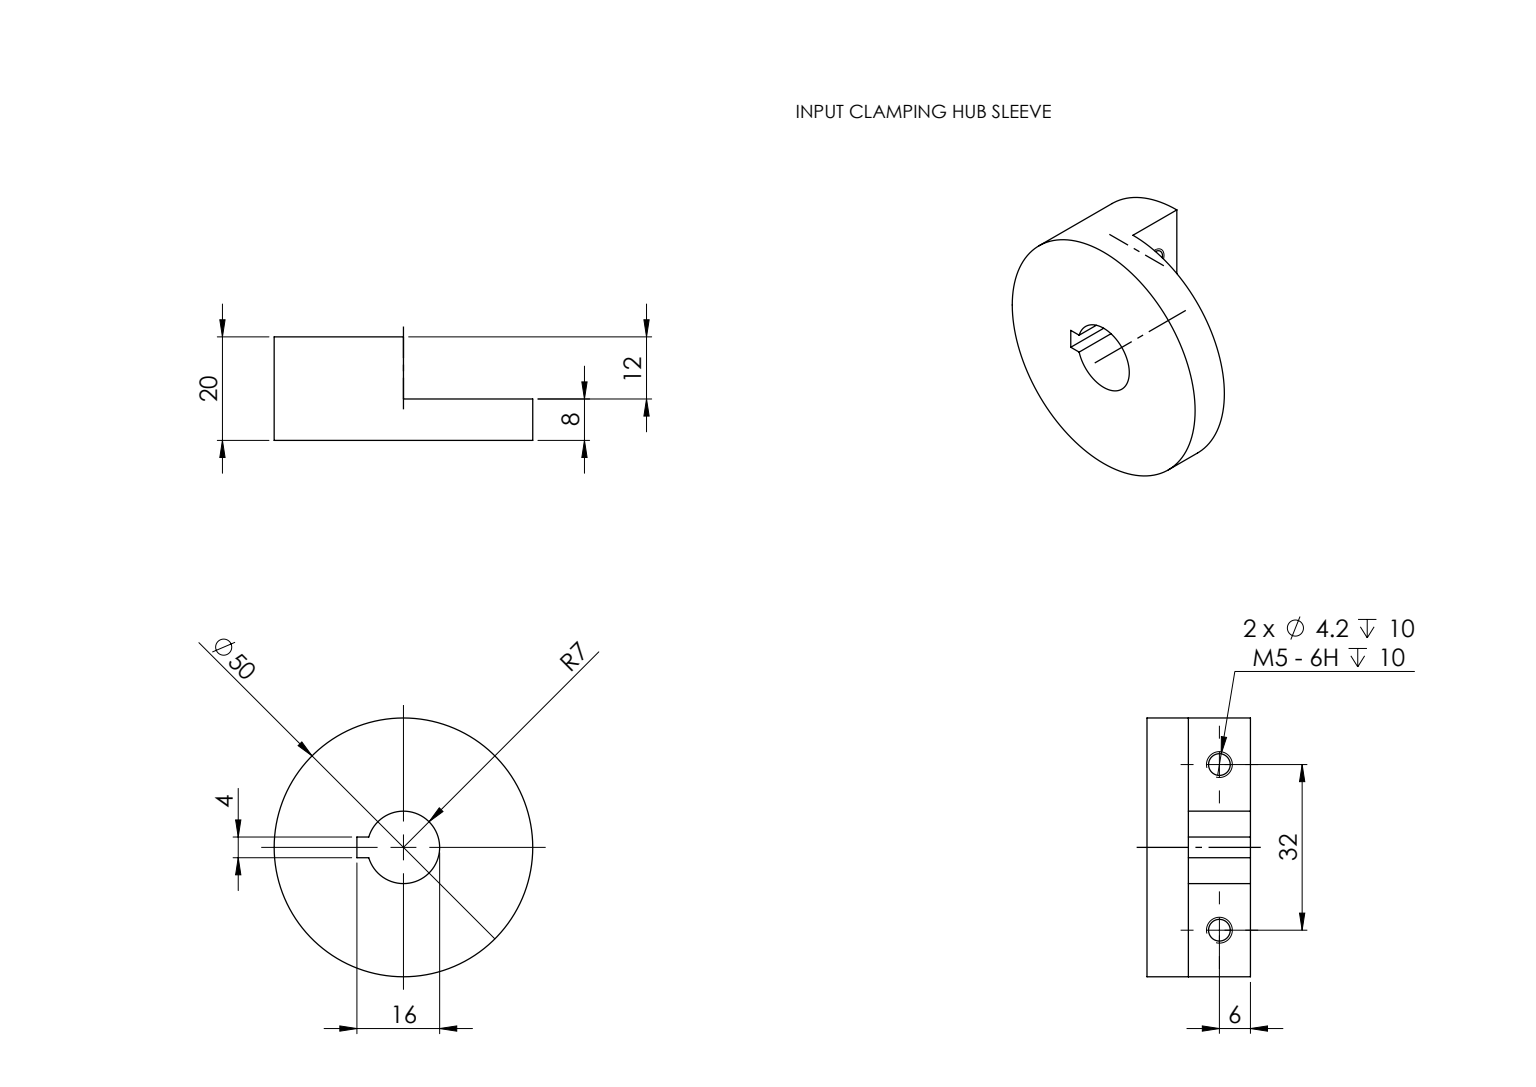
ISO-10303-21;
HEADER;
FILE_DESCRIPTION (('STEP AP214'),
    '1' );
FILE_NAME ('Input Clamping Hub Sleeve.step',
    '2026-10-08T14:09:18',
    ( '' ),
    ( '' ),
    'SwSTEP 2.0',
    'SolidWorks 2026',
    '' );
FILE_SCHEMA (( 'AUTOMOTIVE_DESIGN' ));
ENDSEC;

DATA;
#8=EDGE_CURVE ( 'NONE', #881, #1919, #4427, .T. ) ;
#13=DIRECTION ( 'NONE',  ( -0.000000000000000000, -0.000000000000000000, 1.000000000000000000 ) ) ;
#15=CARTESIAN_POINT ( 'NONE',  ( -6.708203932499367639, 2.000000000000000888, -20.00000000000000000 ) ) ;
#29=DIRECTION ( 'NONE',  ( -0.000000000000000000, -0.000000000000000000, 1.000000000000000000 ) ) ;
#34=FACE_BOUND ( 'NONE', #887, .T. ) ;
#41=LINE ( 'NONE', #2781, #4907 ) ;
#43=DIRECTION ( 'NONE',  ( 1.000000000000000000, -0.000000000000000000, -0.000000000000000000 ) ) ;
#56=DIRECTION ( 'NONE',  ( 0.000000000000000000, 0.000000000000000000, -1.000000000000000000 ) ) ;
#59=ORIENTED_EDGE ( 'NONE', *, *, #2870, .T. ) ;
#63=DIRECTION ( 'NONE',  ( 1.000000000000000000, -0.000000000000000000, 0.000000000000000000 ) ) ;
#66=ORIENTED_EDGE ( 'NONE', *, *, #2378, .T. ) ;
#73=DIRECTION ( 'NONE',  ( 1.000000000000000000, -0.000000000000000000, -0.000000000000000000 ) ) ;
#80=DIRECTION ( 'NONE',  ( -0.000000000000000000, -0.000000000000000000, 1.000000000000000000 ) ) ;
#87=DIRECTION ( 'NONE',  ( 1.357798298438996130E-15, -1.000000000000000000, 0.000000000000000000 ) ) ;
#91=CIRCLE ( 'NONE', #3370, 2.099999999999997868 ) ;
#94=DIRECTION ( 'NONE',  ( -1.000000000000000000, 0.000000000000000000, 0.000000000000000000 ) ) ;
#105=FACE_OUTER_BOUND ( 'NONE', #4278, .T. ) ;
#107=VERTEX_POINT ( 'NONE', #3557 ) ;
#111=CARTESIAN_POINT ( 'NONE',  ( -9.000000000000003553, -1.999999999999999112, -20.00000000000000000 ) ) ;
#117=CARTESIAN_POINT ( 'NONE',  ( 0.000000000000000000, 25.00000000000000000, -20.00000000000000000 ) ) ;
#132=DIRECTION ( 'NONE',  ( 1.000000000000000000, 2.168404344971009361E-16, 0.000000000000000000 ) ) ;
#136=EDGE_LOOP ( 'NONE', ( #1667, #4376 ) ) ;
#140=DIRECTION ( 'NONE',  ( 0.000000000000000000, 0.000000000000000000, -1.000000000000000000 ) ) ;
#147=CARTESIAN_POINT ( 'NONE',  ( 0.000000000000000000, 0.000000000000000000, -20.00000000000000000 ) ) ;
#149=CARTESIAN_POINT ( 'NONE',  ( -9.999999999999975131, -16.00000000000000000, -28.10000000000000142 ) ) ;
#153=VERTEX_POINT ( 'NONE', #3959 ) ;
#157=ORIENTED_EDGE ( 'NONE', *, *, #1693, .F. ) ;
#166=EDGE_CURVE ( 'NONE', #107, #941, #3578, .T. ) ;
#173=VECTOR ( 'NONE', #4086, 1000.000000000000000 ) ;
#208=ADVANCED_FACE ( 'NONE', ( #2082 ), #4946, .F. ) ;
#223=CARTESIAN_POINT ( 'NONE',  ( -7.332110811570578784E-14, -6.999999999999999112, -32.00000000000000000 ) ) ;
#231=CARTESIAN_POINT ( 'NONE',  ( 2.444036937190193033E-14, 6.999999999999999112, -20.00000000000000000 ) ) ;
#240=VERTEX_POINT ( 'NONE', #2913 ) ;
#241=ORIENTED_EDGE ( 'NONE', *, *, #4762, .F. ) ;
#243=LINE ( 'NONE', #1762, #4071 ) ;
#248=LINE ( 'NONE', #4070, #1913 ) ;
#259=DIRECTION ( 'NONE',  ( 0.000000000000000000, 0.000000000000000000, -1.000000000000000000 ) ) ;
#270=FACE_OUTER_BOUND ( 'NONE', #2121, .T. ) ;
#275=MECHANICAL_DESIGN_GEOMETRIC_PRESENTATION_REPRESENTATION('',(#1381),#2264);
#281=DIRECTION ( 'NONE',  ( 0.000000000000000000, 0.000000000000000000, -1.000000000000000000 ) ) ;
#289=CARTESIAN_POINT ( 'NONE',  ( -9.000000000000003553, -1.999999999999999112, -32.00000000000000000 ) ) ;
#300=DIRECTION ( 'NONE',  ( 0.000000000000000000, 0.000000000000000000, -1.000000000000000000 ) ) ;
#303=ORIENTED_EDGE ( 'NONE', *, *, #3258, .T. ) ;
#305=( GEOMETRIC_REPRESENTATION_CONTEXT ( 3 ) GLOBAL_UNCERTAINTY_ASSIGNED_CONTEXT ( ( #1895 ) ) GLOBAL_UNIT_ASSIGNED_CONTEXT ( ( #3470, #4642, #2320 ) ) REPRESENTATION_CONTEXT ( 'NONE', 'WORKASPACE' ) );
#314=CARTESIAN_POINT ( 'NONE',  ( 0.000000000000000000, 0.000000000000000000, -32.00000000000000000 ) ) ;
#322=EDGE_CURVE ( 'NONE', #2990, #2143, #2362, .T. ) ;
#327=CIRCLE ( 'NONE', #3446, 2.099999999999990763 ) ;
#335=CYLINDRICAL_SURFACE ( 'NONE', #4166, 25.00000000000000000 ) ;
#338=DIRECTION ( 'NONE',  ( 0.000000000000000000, 0.000000000000000000, -1.000000000000000000 ) ) ;
#345=ADVANCED_BREP_SHAPE_REPRESENTATION ( '', ( #3609, #1918 ), #305 ) ;
#349=ORIENTED_EDGE ( 'NONE', *, *, #1643, .T. ) ;
#361=AXIS2_PLACEMENT_3D ( 'NONE', #2287, #1500, #3043 ) ;
#362=EDGE_CURVE ( 'NONE', #1707, #1968, #2444, .T. ) ;
#369=CARTESIAN_POINT ( 'NONE',  ( -9.999999999999975131, -16.00000000000000000, -28.10000000000000142 ) ) ;
#370=CARTESIAN_POINT ( 'NONE',  ( 0.000000000000000000, 0.000000000000000000, -32.00000000000000000 ) ) ;
#377=CARTESIAN_POINT ( 'NONE',  ( -6.708203932499367639, 2.000000000000000888, -12.00000000000000000 ) ) ;
#380=ORIENTED_EDGE ( 'NONE', *, *, #2599, .F. ) ;
#386=ADVANCED_FACE ( 'NONE', ( #971 ), #1098, .T. ) ;
#398=VERTEX_POINT ( 'NONE', #2707 ) ;
#410=DIRECTION ( 'NONE',  ( 0.000000000000000000, 0.000000000000000000, -1.000000000000000000 ) ) ;
#414=CONICAL_SURFACE ( 'NONE', #1848, 2.099999999999997868, 1.029744258676653423 ) ;
#423=CARTESIAN_POINT ( 'NONE',  ( 6.999999999999999112, 0.000000000000000000, -20.00000000000000000 ) ) ;
#432=AXIS2_PLACEMENT_3D ( 'NONE', #1311, #2846, #832 ) ;
#452=PRESENTATION_STYLE_ASSIGNMENT (( #3871 ) ) ;
#459=DIRECTION ( 'NONE',  ( 1.000000000000000000, -0.000000000000000000, -0.000000000000000000 ) ) ;
#465=FILL_AREA_STYLE_COLOUR ( '', #4492 ) ;
#467=VERTEX_POINT ( 'NONE', #1823 ) ;
#468=VERTEX_POINT ( 'NONE', #3797 ) ;
#487=EDGE_CURVE ( 'NONE', #468, #1707, #3426, .T. ) ;
#504=EDGE_LOOP ( 'NONE', ( #3356, #2233, #3231, #687, #2325, #2539 ) ) ;
#506=VECTOR ( 'NONE', #1907, 1000.000000000000000 ) ;
#527=CARTESIAN_POINT ( 'NONE',  ( 0.000000000000000000, -1.999999999999999112, -12.00000000000000000 ) ) ;
#531=CARTESIAN_POINT ( 'NONE',  ( -7.332110811570578784E-14, -6.999999999999999112, -20.00000000000000000 ) ) ;
#532=CARTESIAN_POINT ( 'NONE',  ( -9.999999999999975131, -16.00000000000000000, -26.00000000000000355 ) ) ;
#538=DIRECTION ( 'NONE',  ( 0.000000000000000000, 0.000000000000000000, -1.000000000000000000 ) ) ;
#541=EDGE_CURVE ( 'NONE', #4479, #4279, #1671, .T. ) ;
#557=ORIENTED_EDGE ( 'NONE', *, *, #3777, .T. ) ;
#559=CARTESIAN_POINT ( 'NONE',  ( 0.000000000000000000, 25.00000000000000000, -32.00000000000000000 ) ) ;
#574=PRODUCT_CONTEXT ( 'NONE', #3334, 'mechanical' ) ;
#577=ORIENTED_EDGE ( 'NONE', *, *, #1279, .T. ) ;
#582=CYLINDRICAL_SURFACE ( 'NONE', #2017, 25.00000000000000000 ) ;
#583=AXIS2_PLACEMENT_3D ( 'NONE', #4630, #73, #1654 ) ;
#594=AXIS2_PLACEMENT_3D ( 'NONE', #1405, #1084, #1809 ) ;
#601=EDGE_CURVE ( 'NONE', #4279, #3704, #1126, .T. ) ;
#610=DIRECTION ( 'NONE',  ( 0.5150380749100550437, 0.000000000000000000, -0.8571673007021117785 ) ) ;
#622=ADVANCED_FACE ( 'NONE', ( #3955 ), #3927, .F. ) ;
#623=EDGE_CURVE ( 'NONE', #4219, #2953, #1516, .T. ) ;
#625=FACE_BOUND ( 'NONE', #874, .T. ) ;
#646=EDGE_CURVE ( 'NONE', #1680, #4219, #2359, .T. ) ;
#670=AXIS2_PLACEMENT_3D ( 'NONE', #3868, #3890, #1940 ) ;
#687=ORIENTED_EDGE ( 'NONE', *, *, #2074, .F. ) ;
#711=CARTESIAN_POINT ( 'NONE',  ( 0.000000000000000000, 0.000000000000000000, -20.00000000000000000 ) ) ;
#714=ORIENTED_EDGE ( 'NONE', *, *, #623, .F. ) ;
#723=CARTESIAN_POINT ( 'NONE',  ( -9.000000000000003553, -1.999999999999999112, -32.00000000000000000 ) ) ;
#729=ORIENTED_EDGE ( 'NONE', *, *, #2155, .T. ) ;
#733=LINE ( 'NONE', #3464, #4106 ) ;
#737=AXIS2_PLACEMENT_3D ( 'NONE', #2501, #946, #4021 ) ;
#738=VECTOR ( 'NONE', #1161, 1000.000000000000000 ) ;
#741=CARTESIAN_POINT ( 'NONE',  ( -9.000000000000003553, -1.999999999999999112, -12.00000000000000000 ) ) ;
#744=ORIENTED_EDGE ( 'NONE', *, *, #487, .T. ) ;
#752=DIRECTION ( 'NONE',  ( -1.000000000000000000, 0.000000000000000000, 0.000000000000000000 ) ) ;
#761=EDGE_LOOP ( 'NONE', ( #2798, #4883, #1651, #3117 ) ) ;
#762=DIRECTION ( 'NONE',  ( 1.000000000000000000, -0.000000000000000000, -0.000000000000000000 ) ) ;
#771=CARTESIAN_POINT ( 'NONE',  ( -25.00000000000000000, 3.061616997868383043E-15, -12.00000000000000000 ) ) ;
#779=CARTESIAN_POINT ( 'NONE',  ( -10.00000000000002132, 16.00000000000000000, -26.00000000000000355 ) ) ;
#780=CARTESIAN_POINT ( 'NONE',  ( -10.00000000000002132, 16.00000000000000000, -26.00000000000000355 ) ) ;
#788=CYLINDRICAL_SURFACE ( 'NONE', #4749, 2.099999999999994316 ) ;
#791=CARTESIAN_POINT ( 'NONE',  ( 2.172477277502393807E-14, -16.00000000000000000, -28.09999999999999787 ) ) ;
#792=DIRECTION ( 'NONE',  ( -0.000000000000000000, -0.000000000000000000, 1.000000000000000000 ) ) ;
#814=FILL_AREA_STYLE ('',( #4620 ) ) ;
#818=LINE ( 'NONE', #117, #4015 ) ;
#825=DIRECTION ( 'NONE',  ( 0.000000000000000000, 0.000000000000000000, -1.000000000000000000 ) ) ;
#832=DIRECTION ( 'NONE',  ( 1.000000000000000000, 0.000000000000000000, 0.000000000000000000 ) ) ;
#834=ORIENTED_EDGE ( 'NONE', *, *, #848, .T. ) ;
#841=VECTOR ( 'NONE', #3213, 1000.000000000000000 ) ;
#842=ORIENTED_EDGE ( 'NONE', *, *, #1820, .T. ) ;
#843=ORIENTED_EDGE ( 'NONE', *, *, #4547, .T. ) ;
#844=DIRECTION ( 'NONE',  ( 1.000000000000000000, -0.000000000000000000, -0.000000000000000000 ) ) ;
#848=EDGE_CURVE ( 'NONE', #3754, #468, #3922, .T. ) ;
#853=PRODUCT ( 'Input Clamping Hub Sleeve', 'Input Clamping Hub Sleeve', '', ( #574 ) ) ;
#856=SURFACE_SIDE_STYLE ('',( #2768 ) ) ;
#874=EDGE_LOOP ( 'NONE', ( #4323, #3014, #1256, #4847, #349 ) ) ;
#875=ORIENTED_EDGE ( 'NONE', *, *, #1061, .F. ) ;
#881=VERTEX_POINT ( 'NONE', #3443 ) ;
#883=ORIENTED_EDGE ( 'NONE', *, *, #3777, .F. ) ;
#887=EDGE_LOOP ( 'NONE', ( #157, #875 ) ) ;
#888=AXIS2_PLACEMENT_3D ( 'NONE', #1755, #1321, #140 ) ;
#894=VERTEX_POINT ( 'NONE', #741 ) ;
#898=EDGE_CURVE ( 'NONE', #3704, #1580, #4887, .T. ) ;
#900=AXIS2_PLACEMENT_3D ( 'NONE', #1114, #4163, #1487 ) ;
#912=ORIENTED_EDGE ( 'NONE', *, *, #4390, .F. ) ;
#919=ORIENTED_EDGE ( 'NONE', *, *, #1536, .F. ) ;
#926=ORIENTED_EDGE ( 'NONE', *, *, #2599, .T. ) ;
#930=EDGE_CURVE ( 'NONE', #153, #1150, #1071, .T. ) ;
#941=VERTEX_POINT ( 'NONE', #369 ) ;
#946=DIRECTION ( 'NONE',  ( 1.000000000000000000, -0.000000000000000000, -0.000000000000000000 ) ) ;
#953=ORIENTED_EDGE ( 'NONE', *, *, #646, .F. ) ;
#957=AXIS2_PLACEMENT_3D ( 'NONE', #1468, #300, #2156 ) ;
#971=FACE_OUTER_BOUND ( 'NONE', #761, .T. ) ;
#975=AXIS2_PLACEMENT_3D ( 'NONE', #1315, #3964, #538 ) ;
#976=( LENGTH_UNIT ( ) NAMED_UNIT ( * ) SI_UNIT ( .MILLI., .METRE. ) );
#1001=DIRECTION ( 'NONE',  ( 0.000000000000000000, 0.000000000000000000, -1.000000000000000000 ) ) ;
#1004=( NAMED_UNIT ( * ) SI_UNIT ( $, .STERADIAN. ) SOLID_ANGLE_UNIT ( ) );
#1008=EDGE_LOOP ( 'NONE', ( #4046, #1246, #577 ) ) ;
#1020=EDGE_LOOP ( 'NONE', ( #1983, #557, #59, #4058, #714, #953 ) ) ;
#1045=AXIS2_PLACEMENT_3D ( 'NONE', #711, #2978, #4541 ) ;
#1046=LINE ( 'NONE', #2578, #4876 ) ;
#1052=AXIS2_PLACEMENT_3D ( 'NONE', #4364, #259, #3986 ) ;
#1061=EDGE_CURVE ( 'NONE', #1150, #2856, #327, .T. ) ;
#1068=CIRCLE ( 'NONE', #3623, 6.999999999999999112 ) ;
#1071=LINE ( 'NONE', #2271, #2733 ) ;
#1084=DIRECTION ( 'NONE',  ( 0.000000000000000000, 0.000000000000000000, -1.000000000000000000 ) ) ;
#1092=CYLINDRICAL_SURFACE ( 'NONE', #900, 6.999999999999999112 ) ;
#1093=DIRECTION ( 'NONE',  ( -0.000000000000000000, -0.000000000000000000, 1.000000000000000000 ) ) ;
#1098=PLANE ( 'NONE',  #1638 ) ;
#1114=CARTESIAN_POINT ( 'NONE',  ( 0.000000000000000000, 0.000000000000000000, -20.00000000000000000 ) ) ;
#1115=DIRECTION ( 'NONE',  ( 1.000000000000000000, 0.000000000000000000, 0.000000000000000000 ) ) ;
#1119=ORIENTED_EDGE ( 'NONE', *, *, #4580, .F. ) ;
#1125=ORIENTED_EDGE ( 'NONE', *, *, #3211, .T. ) ;
#1126=CIRCLE ( 'NONE', #4884, 6.999999999999999112 ) ;
#1127=CONICAL_SURFACE ( 'NONE', #3765, 2.099999999999997868, 1.029744258676653423 ) ;
#1133=EDGE_LOOP ( 'NONE', ( #1119, #2771, #3567, #1730 ) ) ;
#1146=CARTESIAN_POINT ( 'NONE',  ( 0.000000000000000000, 0.000000000000000000, 0.000000000000000000 ) ) ;
#1150=VERTEX_POINT ( 'NONE', #3180 ) ;
#1159=DIRECTION ( 'NONE',  ( 0.000000000000000000, 0.000000000000000000, -1.000000000000000000 ) ) ;
#1160=CARTESIAN_POINT ( 'NONE',  ( 2.302289838212012812E-14, -16.00000000000000000, -26.00000000000000355 ) ) ;
#1161=DIRECTION ( 'NONE',  ( -0.000000000000000000, -0.000000000000000000, 1.000000000000000000 ) ) ;
#1181=PRODUCT_DEFINITION ( 'UNKNOWN', '', #4711, #3035 ) ;
#1183=CYLINDRICAL_SURFACE ( 'NONE', #4656, 2.099999999999994316 ) ;
#1185=LINE ( 'NONE', #1931, #738 ) ;
#1193=ORIENTED_EDGE ( 'NONE', *, *, #2053, .T. ) ;
#1198=ORIENTED_EDGE ( 'NONE', *, *, #2102, .T. ) ;
#1200=DIRECTION ( 'NONE',  ( -1.000000000000000000, 0.000000000000000000, 0.000000000000000000 ) ) ;
#1222=VECTOR ( 'NONE', #4199, 1000.000000000000000 ) ;
#1231=ORIENTED_EDGE ( 'NONE', *, *, #1820, .F. ) ;
#1235=FILL_AREA_STYLE ('',( #465 ) ) ;
#1243=CARTESIAN_POINT ( 'NONE',  ( 0.000000000000000000, -25.00000000000000000, -20.00000000000000000 ) ) ;
#1246=ORIENTED_EDGE ( 'NONE', *, *, #166, .T. ) ;
#1252=ORIENTED_EDGE ( 'NONE', *, *, #8, .T. ) ;
#1256=ORIENTED_EDGE ( 'NONE', *, *, #2102, .F. ) ;
#1279=EDGE_CURVE ( 'NONE', #941, #467, #3055, .T. ) ;
#1288=FACE_OUTER_BOUND ( 'NONE', #2721, .T. ) ;
#1290=ORIENTED_EDGE ( 'NONE', *, *, #4955, .T. ) ;
#1311=CARTESIAN_POINT ( 'NONE',  ( 0.000000000000000000, 0.000000000000000000, -20.00000000000000000 ) ) ;
#1315=CARTESIAN_POINT ( 'NONE',  ( -2.042664716792774803E-14, 16.00000000000000000, -26.00000000000000355 ) ) ;
#1317=CARTESIAN_POINT ( 'NONE',  ( -9.000000000000001776, 3.903127820947817540E-15, -20.00000000000000000 ) ) ;
#1321=DIRECTION ( 'NONE',  ( 1.000000000000000000, -0.000000000000000000, -0.000000000000000000 ) ) ;
#1331=SHAPE_DEFINITION_REPRESENTATION ( #1603, #2032 ) ;
#1347=DIRECTION ( 'NONE',  ( -1.000000000000000000, 0.000000000000000000, 0.000000000000000000 ) ) ;
#1350=FACE_OUTER_BOUND ( 'NONE', #1431, .T. ) ;
#1351=VECTOR ( 'NONE', #2106, 1000.000000000000000 ) ;
#1358=CARTESIAN_POINT ( 'NONE',  ( -10.00000000000002132, 16.00000000000000000, -28.10000000000000142 ) ) ;
#1361=EDGE_CURVE ( 'NONE', #3396, #3754, #4924, .T. ) ;
#1379=CARTESIAN_POINT ( 'NONE',  ( 0.000000000000000000, 0.000000000000000000, -32.00000000000000000 ) ) ;
#1381=STYLED_ITEM ( 'NONE', ( #2956 ), #3609 ) ;
#1383=ORIENTED_EDGE ( 'NONE', *, *, #2555, .F. ) ;
#1388=LINE ( 'NONE', #1358, #4480 ) ;
#1401=CARTESIAN_POINT ( 'NONE',  ( -9.999999999999975131, -16.00000000000000000, -26.00000000000000355 ) ) ;
#1405=CARTESIAN_POINT ( 'NONE',  ( 0.000000000000000000, 0.000000000000000000, -12.00000000000000000 ) ) ;
#1406=DIRECTION ( 'NONE',  ( -0.000000000000000000, -0.000000000000000000, 1.000000000000000000 ) ) ;
#1418=CARTESIAN_POINT ( 'NONE',  ( -2.172477277502393807E-14, 16.00000000000000000, -26.00000000000000355 ) ) ;
#1420=ADVANCED_FACE ( 'NONE', ( #2595 ), #335, .T. ) ;
#1431=EDGE_LOOP ( 'NONE', ( #303, #1383, #4360, #843 ) ) ;
#1432=FACE_OUTER_BOUND ( 'NONE', #4960, .T. ) ;
#1435=VECTOR ( 'NONE', #792, 1000.000000000000000 ) ;
#1456=ORIENTED_EDGE ( 'NONE', *, *, #4572, .T. ) ;
#1463=DIRECTION ( 'NONE',  ( -4.336808689942018722E-16, -1.000000000000000000, 0.000000000000000000 ) ) ;
#1468=CARTESIAN_POINT ( 'NONE',  ( 0.000000000000000000, 0.000000000000000000, -20.00000000000000000 ) ) ;
#1483=DIRECTION ( 'NONE',  ( 0.000000000000000000, 0.000000000000000000, -1.000000000000000000 ) ) ;
#1485=ADVANCED_FACE ( 'NONE', ( #3413 ), #414, .F. ) ;
#1487=DIRECTION ( 'NONE',  ( 1.000000000000000000, 0.000000000000000000, 0.000000000000000000 ) ) ;
#1489=ORIENTED_EDGE ( 'NONE', *, *, #166, .F. ) ;
#1497=CARTESIAN_POINT ( 'NONE',  ( -2.042664716792774803E-14, 16.00000000000000000, -28.09999999999999432 ) ) ;
#1500=DIRECTION ( 'NONE',  ( 0.000000000000000000, -1.000000000000000000, 0.000000000000000000 ) ) ;
#1502=DIRECTION ( 'NONE',  ( 0.000000000000000000, 0.000000000000000000, -1.000000000000000000 ) ) ;
#1506=CARTESIAN_POINT ( 'NONE',  ( -9.000000000000001776, 3.903127820947817540E-15, -12.00000000000000000 ) ) ;
#1510=EDGE_CURVE ( 'NONE', #3209, #153, #1610, .T. ) ;
#1516=CIRCLE ( 'NONE', #3756, 25.00000000000000000 ) ;
#1524=LINE ( 'NONE', #3785, #3614 ) ;
#1536=EDGE_CURVE ( 'NONE', #240, #153, #3462, .T. ) ;
#1541=DIRECTION ( 'NONE',  ( -0.000000000000000000, -0.000000000000000000, 1.000000000000000000 ) ) ;
#1560=DIRECTION ( 'NONE',  ( 1.000000000000000000, -0.000000000000000000, -0.000000000000000000 ) ) ;
#1561=DIRECTION ( 'NONE',  ( 0.000000000000000000, 0.000000000000000000, -1.000000000000000000 ) ) ;
#1572=ORIENTED_EDGE ( 'NONE', *, *, #4762, .T. ) ;
#1580=VERTEX_POINT ( 'NONE', #2392 ) ;
#1582=DIRECTION ( 'NONE',  ( 1.000000000000000000, -0.000000000000000000, -0.000000000000000000 ) ) ;
#1584=PLANE ( 'NONE',  #670 ) ;
#1593=AXIS2_PLACEMENT_3D ( 'NONE', #1418, #2954, #3772 ) ;
#1603=PRODUCT_DEFINITION_SHAPE ( 'NONE', 'NONE',  #1181 ) ;
#1610=CIRCLE ( 'NONE', #1928, 2.099999999999997868 ) ;
#1618=PLANE ( 'NONE',  #2668 ) ;
#1619=CARTESIAN_POINT ( 'NONE',  ( -6.708203932499366751, -2.000000000000003553, -32.00000000000000000 ) ) ;
#1626=ORIENTED_EDGE ( 'NONE', *, *, #2155, .F. ) ;
#1634=CARTESIAN_POINT ( 'NONE',  ( -10.00000000000002132, 16.00000000000000000, -23.90000000000000568 ) ) ;
#1635=CARTESIAN_POINT ( 'NONE',  ( -9.999999999999975131, -16.00000000000000000, -23.90000000000000568 ) ) ;
#1638=AXIS2_PLACEMENT_3D ( 'NONE', #4574, #4124, #3744 ) ;
#1642=FACE_OUTER_BOUND ( 'NONE', #2000, .T. ) ;
#1643=EDGE_CURVE ( 'NONE', #4802, #2990, #2695, .T. ) ;
#1651=ORIENTED_EDGE ( 'NONE', *, *, #4474, .F. ) ;
#1654=DIRECTION ( 'NONE',  ( 0.000000000000000000, 0.000000000000000000, -1.000000000000000000 ) ) ;
#1661=MECHANICAL_DESIGN_GEOMETRIC_PRESENTATION_REPRESENTATION('',(#4381),#4055);
#1665=FACE_BOUND ( 'NONE', #136, .T. ) ;
#1667=ORIENTED_EDGE ( 'NONE', *, *, #2961, .F. ) ;
#1671=LINE ( 'NONE', #3523, #2089 ) ;
#1680=VERTEX_POINT ( 'NONE', #559 ) ;
#1682=AXIS2_PLACEMENT_3D ( 'NONE', #532, #459, #2057 ) ;
#1693=EDGE_CURVE ( 'NONE', #2856, #1150, #2104, .T. ) ;
#1699=CIRCLE ( 'NONE', #737, 2.099999999999990763 ) ;
#1701=VECTOR ( 'NONE', #1541, 1000.000000000000000 ) ;
#1707=VERTEX_POINT ( 'NONE', #4770 ) ;
#1710=PLANE ( 'NONE',  #4164 ) ;
#1719=ORIENTED_EDGE ( 'NONE', *, *, #1693, .T. ) ;
#1725=ADVANCED_FACE ( 'NONE', ( #2917 ), #3632, .T. ) ;
#1730=ORIENTED_EDGE ( 'NONE', *, *, #2961, .T. ) ;
#1737=CYLINDRICAL_SURFACE ( 'NONE', #2828, 2.099999999999994316 ) ;
#1749=VECTOR ( 'NONE', #4469, 1000.000000000000000 ) ;
#1752=AXIS2_PLACEMENT_3D ( 'NONE', #3724, #13, #4466 ) ;
#1755=CARTESIAN_POINT ( 'NONE',  ( -9.999999999999975131, -16.00000000000000000, -26.00000000000000355 ) ) ;
#1762=CARTESIAN_POINT ( 'NONE',  ( 25.00000000000000000, 0.000000000000000000, -20.00000000000000000 ) ) ;
#1763=VECTOR ( 'NONE', #80, 1000.000000000000000 ) ;
#1766=EDGE_LOOP ( 'NONE', ( #380, #3790, #3447, #3166 ) ) ;
#1785=CARTESIAN_POINT ( 'NONE',  ( -9.999999999999975131, -16.00000000000000000, -26.00000000000000355 ) ) ;
#1809=DIRECTION ( 'NONE',  ( -1.000000000000000000, 0.000000000000000000, 0.000000000000000000 ) ) ;
#1820=EDGE_CURVE ( 'NONE', #467, #941, #3375, .T. ) ;
#1823=CARTESIAN_POINT ( 'NONE',  ( -9.999999999999975131, -16.00000000000000000, -23.90000000000000568 ) ) ;
#1826=DIRECTION ( 'NONE',  ( 1.000000000000000000, -0.000000000000000000, -0.000000000000000000 ) ) ;
#1833=ORIENTED_EDGE ( 'NONE', *, *, #1510, .F. ) ;
#1848=AXIS2_PLACEMENT_3D ( 'NONE', #1785, #1560, #410 ) ;
#1854=DIRECTION ( 'NONE',  ( 1.000000000000000000, -0.000000000000000000, -0.000000000000000000 ) ) ;
#1861=DIRECTION ( 'NONE',  ( 1.000000000000000000, 0.000000000000000000, 0.000000000000000000 ) ) ;
#1895=UNCERTAINTY_MEASURE_WITH_UNIT (LENGTH_MEASURE( 1.000000000000000082E-05 ), #3470, 'distance_accuracy_value', 'NONE');
#1907=DIRECTION ( 'NONE',  ( 0.5150380749100550437, 1.049727191138617956E-16, 0.8571673007021117785 ) ) ;
#1913=VECTOR ( 'NONE', #3743, 1000.000000000000000 ) ;
#1918=AXIS2_PLACEMENT_3D ( 'NONE', #1146, #2700, #1115 ) ;
#1919=VERTEX_POINT ( 'NONE', #771 ) ;
#1928=AXIS2_PLACEMENT_3D ( 'NONE', #779, #1582, #56 ) ;
#1931=CARTESIAN_POINT ( 'NONE',  ( 6.999999999999999112, 0.000000000000000000, -20.00000000000000000 ) ) ;
#1932=ORIENTED_EDGE ( 'NONE', *, *, #4474, .T. ) ;
#1933=CIRCLE ( 'NONE', #4653, 25.00000000000000000 ) ;
#1935=EDGE_CURVE ( 'NONE', #3401, #3396, #4280, .T. ) ;
#1940=DIRECTION ( 'NONE',  ( 1.357798298438996130E-15, -1.000000000000000000, 0.000000000000000000 ) ) ;
#1948=DIRECTION ( 'NONE',  ( 1.000000000000000000, -0.000000000000000000, -0.000000000000000000 ) ) ;
#1968=VERTEX_POINT ( 'NONE', #2083 ) ;
#1977=ORIENTED_EDGE ( 'NONE', *, *, #4367, .F. ) ;
#1983=ORIENTED_EDGE ( 'NONE', *, *, #3211, .F. ) ;
#2000=EDGE_LOOP ( 'NONE', ( #1572, #3081, #2766, #1193 ) ) ;
#2017=AXIS2_PLACEMENT_3D ( 'NONE', #2890, #4404, #3193 ) ;
#2024=AXIS2_PLACEMENT_3D ( 'NONE', #1401, #1826, #2936 ) ;
#2029=AXIS2_PLACEMENT_3D ( 'NONE', #370, #3373, #4543 ) ;
#2032=SHAPE_REPRESENTATION ( 'Input Clamping Hub Sleeve', ( #1918 ), #305 ) ;
#2053=EDGE_CURVE ( 'NONE', #468, #1580, #3671, .T. ) ;
#2055=CARTESIAN_POINT ( 'NONE',  ( -10.00000000000002132, 16.00000000000000000, -28.10000000000000142 ) ) ;
#2057=DIRECTION ( 'NONE',  ( 0.000000000000000000, 0.000000000000000000, -1.000000000000000000 ) ) ;
#2062=FACE_OUTER_BOUND ( 'NONE', #504, .T. ) ;
#2066=EDGE_CURVE ( 'NONE', #4479, #398, #4900, .T. ) ;
#2074=EDGE_CURVE ( 'NONE', #398, #2990, #3445, .T. ) ;
#2082=FACE_OUTER_BOUND ( 'NONE', #2337, .T. ) ;
#2083=CARTESIAN_POINT ( 'NONE',  ( -25.00000000000000000, 3.061616997868383043E-15, -32.00000000000000000 ) ) ;
#2089=VECTOR ( 'NONE', #2785, 1000.000000000000000 ) ;
#2102=EDGE_CURVE ( 'NONE', #894, #2727, #2758, .T. ) ;
#2104=CIRCLE ( 'NONE', #975, 2.099999999999990763 ) ;
#2106=DIRECTION ( 'NONE',  ( 4.073394895316987600E-15, -1.000000000000000000, 0.000000000000000000 ) ) ;
#2121=EDGE_LOOP ( 'NONE', ( #241, #4188, #2234, #1626, #4386, #1456 ) ) ;
#2128=FACE_OUTER_BOUND ( 'NONE', #4827, .T. ) ;
#2143=VERTEX_POINT ( 'NONE', #2832 ) ;
#2155=EDGE_CURVE ( 'NONE', #4219, #4279, #818, .T. ) ;
#2156=DIRECTION ( 'NONE',  ( -1.000000000000000000, 0.000000000000000000, 0.000000000000000000 ) ) ;
#2160=ADVANCED_FACE ( 'NONE', ( #1665, #1642 ), #1618, .F. ) ;
#2194=DIRECTION ( 'NONE',  ( 1.000000000000000000, -0.000000000000000000, -0.000000000000000000 ) ) ;
#2209=DIRECTION ( 'NONE',  ( -0.000000000000000000, -0.000000000000000000, 1.000000000000000000 ) ) ;
#2219=PLANE ( 'NONE',  #2995 ) ;
#2231=CARTESIAN_POINT ( 'NONE',  ( -9.000000000000001776, 2.000000000000000000, -32.00000000000000000 ) ) ;
#2233=ORIENTED_EDGE ( 'NONE', *, *, #4390, .T. ) ;
#2234=ORIENTED_EDGE ( 'NONE', *, *, #601, .F. ) ;
#2253=EDGE_CURVE ( 'NONE', #240, #3209, #1388, .T. ) ;
#2264=( GEOMETRIC_REPRESENTATION_CONTEXT ( 3 ) GLOBAL_UNCERTAINTY_ASSIGNED_CONTEXT ( ( #4545 ) ) GLOBAL_UNIT_ASSIGNED_CONTEXT ( ( #976, #3281, #1004 ) ) REPRESENTATION_CONTEXT ( 'NONE', 'WORKASPACE' ) );
#2266=CARTESIAN_POINT ( 'NONE',  ( -10.00000000000002132, 16.00000000000000000, -26.00000000000000355 ) ) ;
#2271=CARTESIAN_POINT ( 'NONE',  ( -2.172477277502393807E-14, 16.00000000000000000, -23.90000000000000924 ) ) ;
#2287=CARTESIAN_POINT ( 'NONE',  ( 0.000000000000000000, -1.999999999999999112, -20.00000000000000000 ) ) ;
#2313=LINE ( 'NONE', #111, #1763 ) ;
#2320=( NAMED_UNIT ( * ) SI_UNIT ( $, .STERADIAN. ) SOLID_ANGLE_UNIT ( ) );
#2325=ORIENTED_EDGE ( 'NONE', *, *, #2066, .F. ) ;
#2337=EDGE_LOOP ( 'NONE', ( #1198, #1977, #3574, #2996 ) ) ;
#2348=SURFACE_SIDE_STYLE ('',( #4930 ) ) ;
#2359=LINE ( 'NONE', #4277, #1435 ) ;
#2362=CIRCLE ( 'NONE', #4759, 6.999999999999999112 ) ;
#2371=FACE_OUTER_BOUND ( 'NONE', #3969, .T. ) ;
#2378=EDGE_CURVE ( 'NONE', #1707, #2498, #3735, .T. ) ;
#2392=CARTESIAN_POINT ( 'NONE',  ( -3.666055405785289392E-14, -6.999999999999999112, -20.00000000000000000 ) ) ;
#2420=DIRECTION ( 'NONE',  ( 1.000000000000000000, -0.000000000000000000, -0.000000000000000000 ) ) ;
#2422=AXIS2_PLACEMENT_3D ( 'NONE', #1160, #2690, #4201 ) ;
#2434=CARTESIAN_POINT ( 'NONE',  ( 0.000000000000000000, 0.000000000000000000, -20.00000000000000000 ) ) ;
#2438=ADVANCED_FACE ( 'NONE', ( #3808 ), #1127, .F. ) ;
#2444=CIRCLE ( 'NONE', #3479, 25.00000000000000000 ) ;
#2448=ORIENTED_EDGE ( 'NONE', *, *, #930, .F. ) ;
#2468=( NAMED_UNIT ( * ) PLANE_ANGLE_UNIT ( ) SI_UNIT ( $, .RADIAN. ) );
#2478=ORIENTED_EDGE ( 'NONE', *, *, #4572, .F. ) ;
#2479=VECTOR ( 'NONE', #43, 1000.000000000000000 ) ;
#2498=VERTEX_POINT ( 'NONE', #1243 ) ;
#2499=CIRCLE ( 'NONE', #2422, 2.099999999999990763 ) ;
#2501=CARTESIAN_POINT ( 'NONE',  ( 2.302289838212012812E-14, -16.00000000000000000, -26.00000000000000355 ) ) ;
#2510=CONICAL_SURFACE ( 'NONE', #583, 2.099999999999997868, 1.029744258676653423 ) ;
#2515=DIRECTION ( 'NONE',  ( -1.000000000000000000, 0.000000000000000000, -0.000000000000000000 ) ) ;
#2539=ORIENTED_EDGE ( 'NONE', *, *, #541, .T. ) ;
#2555=EDGE_CURVE ( 'NONE', #3396, #894, #2313, .T. ) ;
#2556=EDGE_CURVE ( 'NONE', #107, #467, #4286, .T. ) ;
#2578=CARTESIAN_POINT ( 'NONE',  ( 2.172477277502393807E-14, -16.00000000000000000, -23.90000000000000924 ) ) ;
#2588=CARTESIAN_POINT ( 'NONE',  ( 25.00000000000000000, 0.000000000000000000, -20.00000000000000000 ) ) ;
#2595=FACE_OUTER_BOUND ( 'NONE', #3374, .T. ) ;
#2599=EDGE_CURVE ( 'NONE', #153, #3209, #91, .T. ) ;
#2630=ORIENTED_EDGE ( 'NONE', *, *, #646, .T. ) ;
#2668=AXIS2_PLACEMENT_3D ( 'NONE', #2801, #4644, #3182 ) ;
#2689=ADVANCED_FACE ( 'NONE', ( #1350 ), #1710, .F. ) ;
#2690=DIRECTION ( 'NONE',  ( 1.000000000000000000, -0.000000000000000000, -0.000000000000000000 ) ) ;
#2695=LINE ( 'NONE', #4206, #3695 ) ;
#2700=DIRECTION ( 'NONE',  ( 0.000000000000000000, 0.000000000000000000, 1.000000000000000000 ) ) ;
#2707=CARTESIAN_POINT ( 'NONE',  ( -6.708203932499367639, 2.000000000000001332, -32.00000000000000000 ) ) ;
#2710=FACE_OUTER_BOUND ( 'NONE', #3156, .T. ) ;
#2714=ADVANCED_FACE ( 'NONE', ( #3248 ), #582, .T. ) ;
#2718=DIRECTION ( 'NONE',  ( 1.357798298438996130E-15, -1.000000000000000000, 0.000000000000000000 ) ) ;
#2721=EDGE_LOOP ( 'NONE', ( #4798, #3582 ) ) ;
#2727=VERTEX_POINT ( 'NONE', #4743 ) ;
#2733=VECTOR ( 'NONE', #762, 1000.000000000000000 ) ;
#2735=VECTOR ( 'NONE', #3463, 1000.000000000000000 ) ;
#2752=ORIENTED_EDGE ( 'NONE', *, *, #1510, .T. ) ;
#2758=LINE ( 'NONE', #527, #2831 ) ;
#2762=VERTEX_POINT ( 'NONE', #4056 ) ;
#2766=ORIENTED_EDGE ( 'NONE', *, *, #487, .F. ) ;
#2768=SURFACE_STYLE_FILL_AREA ( #1235 ) ;
#2771=ORIENTED_EDGE ( 'NONE', *, *, #1279, .F. ) ;
#2777=ADVANCED_FACE ( 'NONE', ( #625, #1288 ), #4384, .F. ) ;
#2781=CARTESIAN_POINT ( 'NONE',  ( -25.00000000000000000, 3.061616997868383043E-15, -20.00000000000000000 ) ) ;
#2785=DIRECTION ( 'NONE',  ( -0.000000000000000000, -0.000000000000000000, 1.000000000000000000 ) ) ;
#2798=ORIENTED_EDGE ( 'NONE', *, *, #1643, .F. ) ;
#2799=ORIENTED_EDGE ( 'NONE', *, *, #4367, .T. ) ;
#2801=CARTESIAN_POINT ( 'NONE',  ( -7.332110811570578784E-14, -6.999999999999999112, -32.00000000000000000 ) ) ;
#2806=CARTESIAN_POINT ( 'NONE',  ( -9.000000000000001776, 2.000000000000000000, -12.00000000000000000 ) ) ;
#2820=VECTOR ( 'NONE', #4894, 1000.000000000000000 ) ;
#2828=AXIS2_PLACEMENT_3D ( 'NONE', #3301, #4829, #4439 ) ;
#2831=VECTOR ( 'NONE', #63, 1000.000000000000000 ) ;
#2832=CARTESIAN_POINT ( 'NONE',  ( 6.999999999999999112, 0.000000000000000000, -12.00000000000000000 ) ) ;
#2846=DIRECTION ( 'NONE',  ( -0.000000000000000000, -0.000000000000000000, 1.000000000000000000 ) ) ;
#2848=ORIENTED_EDGE ( 'NONE', *, *, #4669, .F. ) ;
#2854=DIRECTION ( 'NONE',  ( -1.000000000000000000, 4.336808689942018722E-16, 0.000000000000000000 ) ) ;
#2856=VERTEX_POINT ( 'NONE', #1497 ) ;
#2870=EDGE_CURVE ( 'NONE', #1919, #881, #1933, .T. ) ;
#2890=CARTESIAN_POINT ( 'NONE',  ( 0.000000000000000000, 0.000000000000000000, -20.00000000000000000 ) ) ;
#2913=CARTESIAN_POINT ( 'NONE',  ( -11.26180729995789775, 15.99999999999999645, -26.00000000000000355 ) ) ;
#2917=FACE_OUTER_BOUND ( 'NONE', #4628, .T. ) ;
#2934=ORIENTED_EDGE ( 'NONE', *, *, #2253, .F. ) ;
#2936=DIRECTION ( 'NONE',  ( 0.000000000000000000, 0.000000000000000000, -1.000000000000000000 ) ) ;
#2953=VERTEX_POINT ( 'NONE', #2588 ) ;
#2954=DIRECTION ( 'NONE',  ( 1.000000000000000000, -0.000000000000000000, -0.000000000000000000 ) ) ;
#2956=PRESENTATION_STYLE_ASSIGNMENT (( #4398 ) ) ;
#2961=EDGE_CURVE ( 'Edge1', #2762, #4063, #2499, .T. ) ;
#2978=DIRECTION ( 'NONE',  ( 0.000000000000000000, 0.000000000000000000, -1.000000000000000000 ) ) ;
#2984=CARTESIAN_POINT ( 'NONE',  ( -9.000000000000001776, 2.000000000000000000, -20.00000000000000000 ) ) ;
#2990=VERTEX_POINT ( 'NONE', #377 ) ;
#2995=AXIS2_PLACEMENT_3D ( 'NONE', #4848, #338, #4926 ) ;
#2996=ORIENTED_EDGE ( 'NONE', *, *, #2555, .T. ) ;
#3014=ORIENTED_EDGE ( 'NONE', *, *, #3941, .T. ) ;
#3035=PRODUCT_DEFINITION_CONTEXT ( 'detailed design', #4189, 'design' ) ;
#3037=DIRECTION ( 'NONE',  ( 1.000000000000000000, -0.000000000000000000, -0.000000000000000000 ) ) ;
#3043=DIRECTION ( 'NONE',  ( 0.000000000000000000, 0.000000000000000000, -1.000000000000000000 ) ) ;
#3045=CARTESIAN_POINT ( 'NONE',  ( 0.000000000000000000, 0.000000000000000000, -20.00000000000000000 ) ) ;
#3055=CIRCLE ( 'NONE', #888, 2.099999999999997868 ) ;
#3081=ORIENTED_EDGE ( 'NONE', *, *, #2378, .F. ) ;
#3092=CARTESIAN_POINT ( 'NONE',  ( -9.000000000000001776, 2.000000000000000000, -32.00000000000000000 ) ) ;
#3102=ORIENTED_EDGE ( 'NONE', *, *, #1935, .T. ) ;
#3104=CARTESIAN_POINT ( 'NONE',  ( -2.042664716792774803E-14, 16.00000000000000000, -26.00000000000000355 ) ) ;
#3109=DIRECTION ( 'NONE',  ( 0.000000000000000000, 0.000000000000000000, -1.000000000000000000 ) ) ;
#3117=ORIENTED_EDGE ( 'NONE', *, *, #2074, .T. ) ;
#3156=EDGE_LOOP ( 'NONE', ( #1231, #4041, #4588, #2848 ) ) ;
#3160=DIRECTION ( 'NONE',  ( 0.000000000000000000, 0.000000000000000000, -1.000000000000000000 ) ) ;
#3163=CLOSED_SHELL ( 'NONE', ( #4542, #3566, #3390, #622, #3597, #2714, #1420, #3958, #2777, #208, #2689, #386, #3241, #4075, #2160, #1725, #1485, #3768, #2438, #3205 ) ) ;
#3166=ORIENTED_EDGE ( 'NONE', *, *, #3451, .F. ) ;
#3180=CARTESIAN_POINT ( 'NONE',  ( -2.042664716792774803E-14, 16.00000000000000000, -23.90000000000001279 ) ) ;
#3182=DIRECTION ( 'NONE',  ( 4.073394895316987600E-15, -1.000000000000000000, 0.000000000000000000 ) ) ;
#3186=EDGE_CURVE ( 'Edge1', #4063, #2762, #1699, .T. ) ;
#3193=DIRECTION ( 'NONE',  ( 1.000000000000000000, 0.000000000000000000, 0.000000000000000000 ) ) ;
#3205=ADVANCED_FACE ( 'NONE', ( #2128 ), #1737, .F. ) ;
#3209=VERTEX_POINT ( 'NONE', #2055 ) ;
#3211=EDGE_CURVE ( 'NONE', #1968, #1680, #3455, .T. ) ;
#3213=DIRECTION ( 'NONE',  ( 0.5150380749100550437, 0.000000000000000000, -0.8571673007021117785 ) ) ;
#3225=ORIENTED_EDGE ( 'NONE', *, *, #362, .F. ) ;
#3231=ORIENTED_EDGE ( 'NONE', *, *, #322, .F. ) ;
#3241=ADVANCED_FACE ( 'NONE', ( #1432 ), #1092, .F. ) ;
#3248=FACE_OUTER_BOUND ( 'NONE', #1020, .T. ) ;
#3258=EDGE_CURVE ( 'NONE', #4802, #894, #3696, .T. ) ;
#3281=( NAMED_UNIT ( * ) PLANE_ANGLE_UNIT ( ) SI_UNIT ( $, .RADIAN. ) );
#3285=DIRECTION ( 'NONE',  ( -4.336808689942018722E-16, -1.000000000000000000, 0.000000000000000000 ) ) ;
#3299=AXIS2_PLACEMENT_3D ( 'NONE', #314, #4929, #3325 ) ;
#3301=CARTESIAN_POINT ( 'NONE',  ( -2.172477277502393807E-14, 16.00000000000000000, -26.00000000000000355 ) ) ;
#3308=CYLINDRICAL_SURFACE ( 'NONE', #1593, 2.099999999999994316 ) ;
#3325=DIRECTION ( 'NONE',  ( -1.000000000000000000, 0.000000000000000000, 0.000000000000000000 ) ) ;
#3330=FACE_OUTER_BOUND ( 'NONE', #1766, .T. ) ;
#3334=APPLICATION_CONTEXT ( 'automotive_design' ) ;
#3341=CARTESIAN_POINT ( 'NONE',  ( 0.000000000000000000, -25.00000000000000000, -32.00000000000000000 ) ) ;
#3342=DIRECTION ( 'NONE',  ( -1.000000000000000000, 0.000000000000000000, 0.000000000000000000 ) ) ;
#3350=LINE ( 'NONE', #2984, #1749 ) ;
#3356=ORIENTED_EDGE ( 'NONE', *, *, #601, .T. ) ;
#3370=AXIS2_PLACEMENT_3D ( 'NONE', #780, #2420, #1561 ) ;
#3373=DIRECTION ( 'NONE',  ( -0.000000000000000000, -0.000000000000000000, 1.000000000000000000 ) ) ;
#3374=EDGE_LOOP ( 'NONE', ( #883, #3225, #66, #2478, #1290, #1252 ) ) ;
#3375=CIRCLE ( 'NONE', #2024, 2.099999999999997868 ) ;
#3376=DIRECTION ( 'NONE',  ( 1.000000000000000000, -0.000000000000000000, -0.000000000000000000 ) ) ;
#3390=ADVANCED_FACE ( 'NONE', ( #2710 ), #1183, .F. ) ;
#3396=VERTEX_POINT ( 'NONE', #723 ) ;
#3401=VERTEX_POINT ( 'NONE', #2231 ) ;
#3404=CARTESIAN_POINT ( 'NONE',  ( -7.332110811570578784E-14, -6.999999999999999112, -32.00000000000000000 ) ) ;
#3413=FACE_OUTER_BOUND ( 'NONE', #1008, .T. ) ;
#3426=LINE ( 'NONE', #3404, #3839 ) ;
#3443=CARTESIAN_POINT ( 'NONE',  ( 25.00000000000000000, 0.000000000000000000, -12.00000000000000000 ) ) ;
#3445=LINE ( 'NONE', #15, #1701 ) ;
#3446=AXIS2_PLACEMENT_3D ( 'NONE', #3104, #844, #4269 ) ;
#3447=ORIENTED_EDGE ( 'NONE', *, *, #1061, .T. ) ;
#3451=EDGE_CURVE ( 'NONE', #3209, #2856, #3824, .T. ) ;
#3454=ORIENTED_EDGE ( 'NONE', *, *, #1536, .T. ) ;
#3455=CIRCLE ( 'NONE', #3299, 25.00000000000000000 ) ;
#3462=LINE ( 'NONE', #1634, #506 ) ;
#3463=DIRECTION ( 'NONE',  ( 0.5150380749100550437, 1.049727191138617956E-16, 0.8571673007021117785 ) ) ;
#3464=CARTESIAN_POINT ( 'NONE',  ( 0.000000000000000000, 25.00000000000000000, -32.00000000000000000 ) ) ;
#3470=( LENGTH_UNIT ( ) NAMED_UNIT ( * ) SI_UNIT ( .MILLI., .METRE. ) );
#3479=AXIS2_PLACEMENT_3D ( 'NONE', #3702, #281, #1347 ) ;
#3486=CARTESIAN_POINT ( 'NONE',  ( -2.172477277502393807E-14, 16.00000000000000000, -28.09999999999999787 ) ) ;
#3493=CARTESIAN_POINT ( 'NONE',  ( 2.302289838212012812E-14, -16.00000000000000000, -23.90000000000001279 ) ) ;
#3523=CARTESIAN_POINT ( 'NONE',  ( 2.444036937190193033E-14, 6.999999999999999112, -32.00000000000000000 ) ) ;
#3538=VECTOR ( 'NONE', #1463, 1000.000000000000000 ) ;
#3557=CARTESIAN_POINT ( 'NONE',  ( -11.26180729995785157, -16.00000000000000355, -26.00000000000000355 ) ) ;
#3563=DIRECTION ( 'NONE',  ( 0.000000000000000000, 0.000000000000000000, -1.000000000000000000 ) ) ;
#3566=ADVANCED_FACE ( 'NONE', ( #105 ), #2510, .F. ) ;
#3567=ORIENTED_EDGE ( 'NONE', *, *, #4669, .T. ) ;
#3568=ORIENTED_EDGE ( 'NONE', *, *, #4039, .T. ) ;
#3574=ORIENTED_EDGE ( 'NONE', *, *, #1361, .F. ) ;
#3578=LINE ( 'NONE', #149, #841 ) ;
#3582=ORIENTED_EDGE ( 'NONE', *, *, #2870, .F. ) ;
#3597=ADVANCED_FACE ( 'NONE', ( #2062 ), #4255, .F. ) ;
#3609=MANIFOLD_SOLID_BREP ( 'M5 Tapped Hole1', #3163 ) ;
#3614=VECTOR ( 'NONE', #29, 1000.000000000000000 ) ;
#3623=AXIS2_PLACEMENT_3D ( 'NONE', #3662, #1483, #3342 ) ;
#3632=PLANE ( 'NONE',  #4168 ) ;
#3651=EDGE_LOOP ( 'NONE', ( #919, #4633, #2752 ) ) ;
#3662=CARTESIAN_POINT ( 'NONE',  ( 0.000000000000000000, 0.000000000000000000, -12.00000000000000000 ) ) ;
#3666=CIRCLE ( 'NONE', #957, 25.00000000000000000 ) ;
#3671=LINE ( 'NONE', #223, #3699 ) ;
#3695=VECTOR ( 'NONE', #132, 1000.000000000000000 ) ;
#3696=LINE ( 'NONE', #1506, #3538 ) ;
#3699=VECTOR ( 'NONE', #4212, 1000.000000000000000 ) ;
#3702=CARTESIAN_POINT ( 'NONE',  ( 0.000000000000000000, 0.000000000000000000, -32.00000000000000000 ) ) ;
#3704=VERTEX_POINT ( 'NONE', #423 ) ;
#3724=CARTESIAN_POINT ( 'NONE',  ( 0.000000000000000000, 0.000000000000000000, -32.00000000000000000 ) ) ;
#3735=LINE ( 'NONE', #3341, #2820 ) ;
#3737=COLOUR_RGB ( '', 0.08235294, 0.09019608, 0.10196078) ;
#3743=DIRECTION ( 'NONE',  ( -1.000000000000000000, -3.784637517658031179E-16, -0.000000000000000000 ) ) ;
#3744=DIRECTION ( 'NONE',  ( 1.000000000000000000, 2.168404344971009361E-16, 0.000000000000000000 ) ) ;
#3754=VERTEX_POINT ( 'NONE', #1619 ) ;
#3756=AXIS2_PLACEMENT_3D ( 'NONE', #147, #825, #1200 ) ;
#3765=AXIS2_PLACEMENT_3D ( 'NONE', #2266, #2194, #1502 ) ;
#3768=ADVANCED_FACE ( 'NONE', ( #4213 ), #788, .F. ) ;
#3772=DIRECTION ( 'NONE',  ( 0.000000000000000000, 0.000000000000000000, -1.000000000000000000 ) ) ;
#3777=EDGE_CURVE ( 'NONE', #1968, #1919, #41, .T. ) ;
#3785=CARTESIAN_POINT ( 'NONE',  ( -6.708203932499366751, -2.000000000000003553, -20.00000000000000000 ) ) ;
#3790=ORIENTED_EDGE ( 'NONE', *, *, #930, .T. ) ;
#3797=CARTESIAN_POINT ( 'NONE',  ( -7.332110811570578784E-14, -6.999999999999999112, -32.00000000000000000 ) ) ;
#3808=FACE_OUTER_BOUND ( 'NONE', #3651, .T. ) ;
#3824=LINE ( 'NONE', #3486, #4020 ) ;
#3839=VECTOR ( 'NONE', #3851, 1000.000000000000000 ) ;
#3851=DIRECTION ( 'NONE',  ( 4.073394895316987600E-15, -1.000000000000000000, 0.000000000000000000 ) ) ;
#3868=CARTESIAN_POINT ( 'NONE',  ( 0.000000000000000000, 25.00000000000000000, -32.00000000000000000 ) ) ;
#3871=SURFACE_STYLE_USAGE ( .BOTH. , #2348 ) ;
#3880=LINE ( 'NONE', #791, #2479 ) ;
#3887=ORIENTED_EDGE ( 'NONE', *, *, #3451, .T. ) ;
#3890=DIRECTION ( 'NONE',  ( -1.000000000000000000, -1.357798298438996130E-15, 0.000000000000000000 ) ) ;
#3893=( NAMED_UNIT ( * ) SI_UNIT ( $, .STERADIAN. ) SOLID_ANGLE_UNIT ( ) );
#3922=CIRCLE ( 'NONE', #1752, 6.999999999999999112 ) ;
#3927=CONICAL_SURFACE ( 'NONE', #1682, 2.099999999999997868, 1.029744258676653423 ) ;
#3937=ORIENTED_EDGE ( 'NONE', *, *, #2556, .T. ) ;
#3941=EDGE_CURVE ( 'NONE', #2143, #2727, #1068, .T. ) ;
#3955=FACE_OUTER_BOUND ( 'NONE', #4601, .T. ) ;
#3958=ADVANCED_FACE ( 'NONE', ( #270 ), #2219, .T. ) ;
#3959=CARTESIAN_POINT ( 'NONE',  ( -10.00000000000002132, 16.00000000000000000, -23.90000000000000568 ) ) ;
#3962=ORIENTED_EDGE ( 'NONE', *, *, #2053, .F. ) ;
#3964=DIRECTION ( 'NONE',  ( 1.000000000000000000, -0.000000000000000000, -0.000000000000000000 ) ) ;
#3969=EDGE_LOOP ( 'NONE', ( #729, #4820, #4301, #2630 ) ) ;
#3986=DIRECTION ( 'NONE',  ( -1.000000000000000000, 0.000000000000000000, -0.000000000000000000 ) ) ;
#4007=CARTESIAN_POINT ( 'NONE',  ( 0.000000000000000000, 25.00000000000000000, -20.00000000000000000 ) ) ;
#4015=VECTOR ( 'NONE', #87, 1000.000000000000000 ) ;
#4020=VECTOR ( 'NONE', #1854, 1000.000000000000000 ) ;
#4021=DIRECTION ( 'NONE',  ( 0.000000000000000000, 0.000000000000000000, -1.000000000000000000 ) ) ;
#4039=EDGE_CURVE ( 'NONE', #1680, #4479, #733, .T. ) ;
#4041=ORIENTED_EDGE ( 'NONE', *, *, #4580, .T. ) ;
#4046=ORIENTED_EDGE ( 'NONE', *, *, #2556, .F. ) ;
#4055=( GEOMETRIC_REPRESENTATION_CONTEXT ( 3 ) GLOBAL_UNCERTAINTY_ASSIGNED_CONTEXT ( ( #4245 ) ) GLOBAL_UNIT_ASSIGNED_CONTEXT ( ( #4539, #2468, #3893 ) ) REPRESENTATION_CONTEXT ( 'NONE', 'WORKASPACE' ) );
#4056=CARTESIAN_POINT ( 'NONE',  ( 2.302289838212012812E-14, -16.00000000000000000, -28.09999999999999432 ) ) ;
#4058=ORIENTED_EDGE ( 'NONE', *, *, #4955, .F. ) ;
#4063=VERTEX_POINT ( 'NONE', #3493 ) ;
#4070=CARTESIAN_POINT ( 'NONE',  ( -9.000000000000001776, 2.000000000000000000, -32.00000000000000000 ) ) ;
#4071=VECTOR ( 'NONE', #1093, 1000.000000000000000 ) ;
#4075=ADVANCED_FACE ( 'Placement Plane', ( #34, #2371 ), #1584, .F. ) ;
#4086=DIRECTION ( 'NONE',  ( 1.000000000000000000, -1.892318758829013864E-15, 0.000000000000000000 ) ) ;
#4106=VECTOR ( 'NONE', #2718, 1000.000000000000000 ) ;
#4108=CARTESIAN_POINT ( 'NONE',  ( 0.000000000000000000, 0.000000000000000000, -12.00000000000000000 ) ) ;
#4124=DIRECTION ( 'NONE',  ( 2.168404344971009361E-16, -1.000000000000000000, 0.000000000000000000 ) ) ;
#4163=DIRECTION ( 'NONE',  ( -0.000000000000000000, -0.000000000000000000, 1.000000000000000000 ) ) ;
#4164=AXIS2_PLACEMENT_3D ( 'NONE', #1317, #2854, #3285 ) ;
#4166=AXIS2_PLACEMENT_3D ( 'NONE', #3045, #1406, #1861 ) ;
#4167=ORIENTED_EDGE ( 'NONE', *, *, #848, .F. ) ;
#4168=AXIS2_PLACEMENT_3D ( 'NONE', #1379, #3563, #2515 ) ;
#4188=ORIENTED_EDGE ( 'NONE', *, *, #898, .F. ) ;
#4189=APPLICATION_CONTEXT ( 'automotive_design' ) ;
#4199=DIRECTION ( 'NONE',  ( -4.336808689942018722E-16, -1.000000000000000000, 0.000000000000000000 ) ) ;
#4201=DIRECTION ( 'NONE',  ( 0.000000000000000000, 0.000000000000000000, -1.000000000000000000 ) ) ;
#4206=CARTESIAN_POINT ( 'NONE',  ( -4.336808689942023652E-16, 2.000000000000002220, -12.00000000000000000 ) ) ;
#4212=DIRECTION ( 'NONE',  ( -0.000000000000000000, -0.000000000000000000, 1.000000000000000000 ) ) ;
#4213=FACE_OUTER_BOUND ( 'NONE', #1133, .T. ) ;
#4219=VERTEX_POINT ( 'NONE', #4007 ) ;
#4223=CARTESIAN_POINT ( 'NONE',  ( 2.172477277502393807E-14, -16.00000000000000000, -26.00000000000000355 ) ) ;
#4245=UNCERTAINTY_MEASURE_WITH_UNIT (LENGTH_MEASURE( 1.000000000000000082E-05 ), #4539, 'distance_accuracy_value', 'NONE');
#4248=ORIENTED_EDGE ( 'NONE', *, *, #362, .T. ) ;
#4255=CYLINDRICAL_SURFACE ( 'NONE', #432, 6.999999999999999112 ) ;
#4269=DIRECTION ( 'NONE',  ( 0.000000000000000000, 0.000000000000000000, -1.000000000000000000 ) ) ;
#4277=CARTESIAN_POINT ( 'NONE',  ( 0.000000000000000000, 25.00000000000000000, -32.00000000000000000 ) ) ;
#4278=EDGE_LOOP ( 'NONE', ( #2934, #3454, #926 ) ) ;
#4279=VERTEX_POINT ( 'NONE', #231 ) ;
#4280=LINE ( 'NONE', #3092, #1222 ) ;
#4286=LINE ( 'NONE', #1635, #2735 ) ;
#4301=ORIENTED_EDGE ( 'NONE', *, *, #4039, .F. ) ;
#4323=ORIENTED_EDGE ( 'NONE', *, *, #322, .T. ) ;
#4360=ORIENTED_EDGE ( 'NONE', *, *, #1935, .F. ) ;
#4364=CARTESIAN_POINT ( 'NONE',  ( 0.000000000000000000, 0.000000000000000000, -12.00000000000000000 ) ) ;
#4367=EDGE_CURVE ( 'NONE', #3754, #2727, #1524, .T. ) ;
#4376=ORIENTED_EDGE ( 'NONE', *, *, #3186, .F. ) ;
#4377=DIRECTION ( 'NONE',  ( -1.000000000000000000, 0.000000000000000000, 0.000000000000000000 ) ) ;
#4381=STYLED_ITEM ( 'NONE', ( #452 ), #345 ) ;
#4384=PLANE ( 'NONE',  #1052 ) ;
#4386=ORIENTED_EDGE ( 'NONE', *, *, #623, .T. ) ;
#4390=EDGE_CURVE ( 'NONE', #3704, #2143, #1185, .T. ) ;
#4393=LINE ( 'NONE', #531, #1351 ) ;
#4398=SURFACE_STYLE_USAGE ( .BOTH. , #856 ) ;
#4404=DIRECTION ( 'NONE',  ( -0.000000000000000000, -0.000000000000000000, 1.000000000000000000 ) ) ;
#4427=CIRCLE ( 'NONE', #594, 25.00000000000000000 ) ;
#4439=DIRECTION ( 'NONE',  ( 0.000000000000000000, 0.000000000000000000, -1.000000000000000000 ) ) ;
#4461=ORIENTED_EDGE ( 'NONE', *, *, #1361, .T. ) ;
#4466=DIRECTION ( 'NONE',  ( -1.000000000000000000, 0.000000000000000000, 0.000000000000000000 ) ) ;
#4469=DIRECTION ( 'NONE',  ( -0.000000000000000000, -0.000000000000000000, 1.000000000000000000 ) ) ;
#4474=EDGE_CURVE ( 'NONE', #398, #3401, #248, .T. ) ;
#4479=VERTEX_POINT ( 'NONE', #4857 ) ;
#4480=VECTOR ( 'NONE', #610, 1000.000000000000000 ) ;
#4492=COLOUR_RGB ( '', 0.08235294, 0.09019608, 0.10196078) ;
#4507=ORIENTED_EDGE ( 'NONE', *, *, #898, .T. ) ;
#4539=( LENGTH_UNIT ( ) NAMED_UNIT ( * ) SI_UNIT ( .MILLI., .METRE. ) );
#4541=DIRECTION ( 'NONE',  ( -1.000000000000000000, 0.000000000000000000, 0.000000000000000000 ) ) ;
#4542=ADVANCED_FACE ( 'NONE', ( #3330 ), #3308, .F. ) ;
#4543=DIRECTION ( 'NONE',  ( -1.000000000000000000, 0.000000000000000000, 0.000000000000000000 ) ) ;
#4545=UNCERTAINTY_MEASURE_WITH_UNIT (LENGTH_MEASURE( 1.000000000000000082E-05 ), #976, 'distance_accuracy_value', 'NONE');
#4547=EDGE_CURVE ( 'NONE', #3401, #4802, #3350, .T. ) ;
#4552=DIRECTION ( 'NONE',  ( 0.000000000000000000, 0.000000000000000000, -1.000000000000000000 ) ) ;
#4572=EDGE_CURVE ( 'NONE', #2953, #2498, #3666, .T. ) ;
#4574=CARTESIAN_POINT ( 'NONE',  ( -4.336808689942023652E-16, 2.000000000000002220, -20.00000000000000000 ) ) ;
#4580=EDGE_CURVE ( 'NONE', #467, #4063, #1046, .T. ) ;
#4588=ORIENTED_EDGE ( 'NONE', *, *, #3186, .T. ) ;
#4597=ORIENTED_EDGE ( 'NONE', *, *, #3941, .F. ) ;
#4601=EDGE_LOOP ( 'NONE', ( #1489, #3937, #842 ) ) ;
#4620=FILL_AREA_STYLE_COLOUR ( '', #3737 ) ;
#4628=EDGE_LOOP ( 'NONE', ( #4248, #1125, #3568, #4877, #1932, #3102, #4461, #834, #744 ) ) ;
#4630=CARTESIAN_POINT ( 'NONE',  ( -10.00000000000002132, 16.00000000000000000, -26.00000000000000355 ) ) ;
#4633=ORIENTED_EDGE ( 'NONE', *, *, #2253, .T. ) ;
#4642=( NAMED_UNIT ( * ) PLANE_ANGLE_UNIT ( ) SI_UNIT ( $, .RADIAN. ) );
#4644=DIRECTION ( 'NONE',  ( -1.000000000000000000, -4.073394895316987600E-15, 0.000000000000000000 ) ) ;
#4653=AXIS2_PLACEMENT_3D ( 'NONE', #4108, #4552, #752 ) ;
#4656=AXIS2_PLACEMENT_3D ( 'NONE', #4223, #3037, #1159 ) ;
#4669=EDGE_CURVE ( 'NONE', #941, #2762, #3880, .T. ) ;
#4674=CARTESIAN_POINT ( 'NONE',  ( 2.172477277502393807E-14, -16.00000000000000000, -26.00000000000000355 ) ) ;
#4692=SHAPE_REPRESENTATION_RELATIONSHIP ( 'NONE' , 'NONE' ,  #2032, #345 ) ;
#4711=PRODUCT_DEFINITION_FORMATION_WITH_SPECIFIED_SOURCE ( 'ANY', '', #853, .NOT_KNOWN. ) ;
#4743=CARTESIAN_POINT ( 'NONE',  ( -6.708203932499366751, -2.000000000000003553, -12.00000000000000000 ) ) ;
#4749=AXIS2_PLACEMENT_3D ( 'NONE', #4674, #1948, #3160 ) ;
#4759=AXIS2_PLACEMENT_3D ( 'NONE', #4805, #1001, #4377 ) ;
#4762=EDGE_CURVE ( 'NONE', #1580, #2498, #4393, .T. ) ;
#4770=CARTESIAN_POINT ( 'NONE',  ( 0.000000000000000000, -25.00000000000000000, -32.00000000000000000 ) ) ;
#4798=ORIENTED_EDGE ( 'NONE', *, *, #8, .F. ) ;
#4802=VERTEX_POINT ( 'NONE', #2806 ) ;
#4805=CARTESIAN_POINT ( 'NONE',  ( 0.000000000000000000, 0.000000000000000000, -12.00000000000000000 ) ) ;
#4820=ORIENTED_EDGE ( 'NONE', *, *, #541, .F. ) ;
#4827=EDGE_LOOP ( 'NONE', ( #2448, #1833, #3887, #1719 ) ) ;
#4829=DIRECTION ( 'NONE',  ( 1.000000000000000000, -0.000000000000000000, -0.000000000000000000 ) ) ;
#4847=ORIENTED_EDGE ( 'NONE', *, *, #3258, .F. ) ;
#4848=CARTESIAN_POINT ( 'NONE',  ( 0.000000000000000000, 0.000000000000000000, -20.00000000000000000 ) ) ;
#4857=CARTESIAN_POINT ( 'NONE',  ( 2.444036937190193033E-14, 6.999999999999999112, -32.00000000000000000 ) ) ;
#4876=VECTOR ( 'NONE', #3376, 1000.000000000000000 ) ;
#4877=ORIENTED_EDGE ( 'NONE', *, *, #2066, .T. ) ;
#4883=ORIENTED_EDGE ( 'NONE', *, *, #4547, .F. ) ;
#4884=AXIS2_PLACEMENT_3D ( 'NONE', #2434, #3109, #94 ) ;
#4887=CIRCLE ( 'NONE', #1045, 6.999999999999999112 ) ;
#4894=DIRECTION ( 'NONE',  ( -0.000000000000000000, -0.000000000000000000, 1.000000000000000000 ) ) ;
#4900=CIRCLE ( 'NONE', #2029, 6.999999999999999112 ) ;
#4907=VECTOR ( 'NONE', #2209, 1000.000000000000000 ) ;
#4924=LINE ( 'NONE', #289, #173 ) ;
#4926=DIRECTION ( 'NONE',  ( -1.000000000000000000, 0.000000000000000000, -0.000000000000000000 ) ) ;
#4929=DIRECTION ( 'NONE',  ( 0.000000000000000000, 0.000000000000000000, -1.000000000000000000 ) ) ;
#4930=SURFACE_STYLE_FILL_AREA ( #814 ) ;
#4946=PLANE ( 'NONE',  #361 ) ;
#4955=EDGE_CURVE ( 'NONE', #2953, #881, #243, .T. ) ;
#4960=EDGE_LOOP ( 'NONE', ( #912, #4507, #3962, #4167, #2799, #4597 ) ) ;
ENDSEC;
END-ISO-10303-21;
